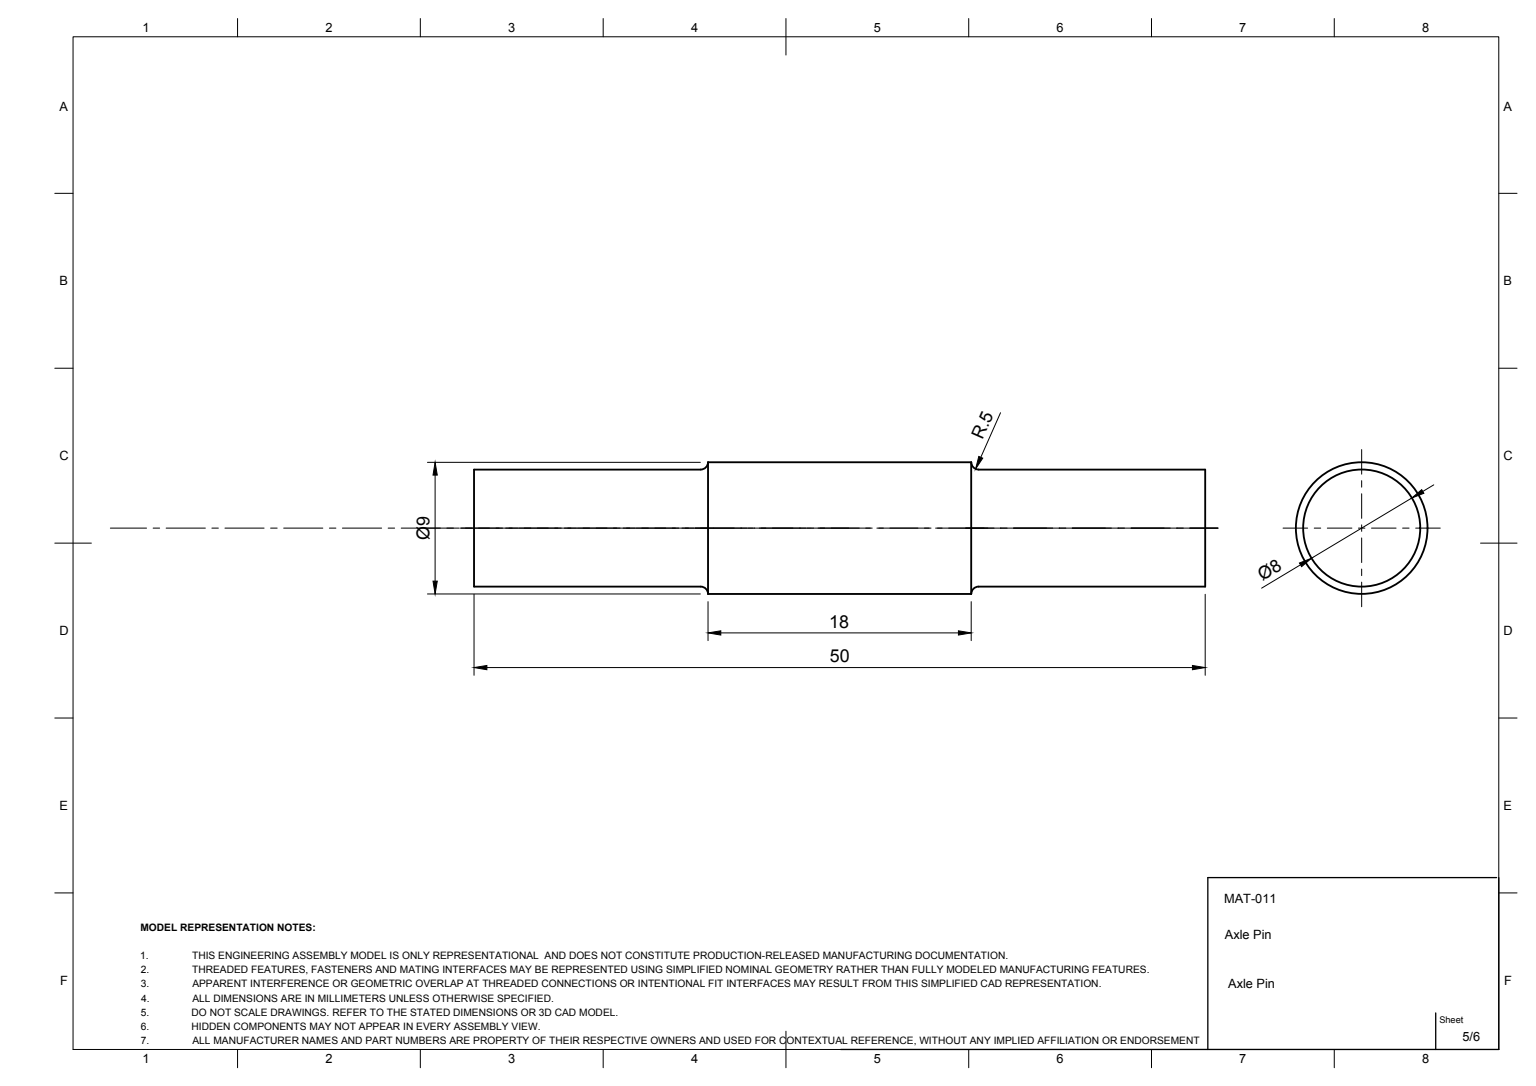
ISO-10303-21;
HEADER;
/* Generated by software containing ST-Developer
 * from STEP Tools, Inc. (www.steptools.com) 
 */

FILE_DESCRIPTION(
/* description */ ('STEP AP214'),
/* implementation_level */ '2;1');

FILE_NAME(
/* name */ 'Axle Pin.step',
/* time_stamp */ '2026-11-14T05:56:09-08:00',
/* author */ (''),
/* organization */ (''),
/* preprocessor_version */ 'ST-DEVELOPER v20.2',
/* originating_system */ 'Autodesk Translation Framework v15.17.0.0',
/* authorisation */ '');

FILE_SCHEMA (('AUTOMOTIVE_DESIGN { 1 0 10303 214 3 1 1 }'));
ENDSEC;

DATA;
#10=MECHANICAL_DESIGN_GEOMETRIC_PRESENTATION_REPRESENTATION('',(#104),#3207);
#92=SHAPE_REPRESENTATION_RELATIONSHIP('SRR','None',#3244,#98);
#98=ADVANCED_BREP_SHAPE_REPRESENTATION('',(#110),#3203);
#104=STYLED_ITEM('',(#3281),#110);
#110=MANIFOLD_SOLID_BREP('Body1',#1282);
#131=PLANE('',#1414);
#132=PLANE('',#1415);
#184=LINE('',#2091,#251);
#185=LINE('',#2093,#252);
#186=LINE('',#2096,#253);
#251=VECTOR('',#1666,4.);
#252=VECTOR('',#1669,4.5);
#253=VECTOR('',#1672,4.);
#290=CYLINDRICAL_SURFACE('',#1409,4.);
#291=CYLINDRICAL_SURFACE('',#1411,4.5);
#292=CYLINDRICAL_SURFACE('',#1412,4.);
#370=FACE_OUTER_BOUND('',#451,.T.);
#371=FACE_OUTER_BOUND('',#452,.T.);
#372=FACE_OUTER_BOUND('',#453,.T.);
#373=FACE_OUTER_BOUND('',#454,.T.);
#374=FACE_OUTER_BOUND('',#455,.T.);
#375=FACE_OUTER_BOUND('',#456,.T.);
#376=FACE_OUTER_BOUND('',#457,.T.);
#451=EDGE_LOOP('',(#965,#966,#967,#968));
#452=EDGE_LOOP('',(#969,#970,#971,#972,#973,#974));
#453=EDGE_LOOP('',(#975,#976,#977,#978,#979));
#454=EDGE_LOOP('',(#980,#981,#982,#983,#984));
#455=EDGE_LOOP('',(#985,#986,#987,#988));
#456=EDGE_LOOP('',(#989));
#457=EDGE_LOOP('',(#990));
#535=CIRCLE('',#1400,4.5);
#536=CIRCLE('',#1401,0.5);
#537=CIRCLE('',#1402,4.);
#538=CIRCLE('',#1404,4.5);
#539=CIRCLE('',#1405,0.5);
#540=CIRCLE('',#1406,4.);
#541=CIRCLE('',#1407,4.);
#542=CIRCLE('',#1408,4.5);
#543=CIRCLE('',#1410,4.);
#544=CIRCLE('',#1413,4.);
#619=VERTEX_POINT('',#2073);
#620=VERTEX_POINT('',#2075);
#621=VERTEX_POINT('',#2079);
#622=VERTEX_POINT('',#2080);
#623=VERTEX_POINT('',#2082);
#624=VERTEX_POINT('',#2084);
#625=VERTEX_POINT('',#2089);
#626=VERTEX_POINT('',#2095);
#746=EDGE_CURVE('',#619,#619,#535,.T.);
#747=EDGE_CURVE('',#619,#620,#536,.T.);
#748=EDGE_CURVE('',#620,#620,#537,.T.);
#749=EDGE_CURVE('',#621,#622,#538,.T.);
#750=EDGE_CURVE('',#622,#623,#539,.T.);
#751=EDGE_CURVE('',#624,#623,#540,.T.);
#752=EDGE_CURVE('',#623,#624,#541,.T.);
#753=EDGE_CURVE('',#622,#621,#542,.T.);
#754=EDGE_CURVE('',#625,#625,#543,.T.);
#755=EDGE_CURVE('',#625,#624,#184,.T.);
#756=EDGE_CURVE('',#621,#619,#185,.T.);
#757=EDGE_CURVE('',#620,#626,#186,.T.);
#758=EDGE_CURVE('',#626,#626,#544,.T.);
#965=ORIENTED_EDGE('',*,*,#746,.F.);
#966=ORIENTED_EDGE('',*,*,#747,.T.);
#967=ORIENTED_EDGE('',*,*,#748,.F.);
#968=ORIENTED_EDGE('',*,*,#747,.F.);
#969=ORIENTED_EDGE('',*,*,#749,.T.);
#970=ORIENTED_EDGE('',*,*,#750,.T.);
#971=ORIENTED_EDGE('',*,*,#751,.F.);
#972=ORIENTED_EDGE('',*,*,#752,.F.);
#973=ORIENTED_EDGE('',*,*,#750,.F.);
#974=ORIENTED_EDGE('',*,*,#753,.T.);
#975=ORIENTED_EDGE('',*,*,#754,.F.);
#976=ORIENTED_EDGE('',*,*,#755,.T.);
#977=ORIENTED_EDGE('',*,*,#751,.T.);
#978=ORIENTED_EDGE('',*,*,#752,.T.);
#979=ORIENTED_EDGE('',*,*,#755,.F.);
#980=ORIENTED_EDGE('',*,*,#749,.F.);
#981=ORIENTED_EDGE('',*,*,#756,.T.);
#982=ORIENTED_EDGE('',*,*,#746,.T.);
#983=ORIENTED_EDGE('',*,*,#756,.F.);
#984=ORIENTED_EDGE('',*,*,#753,.F.);
#985=ORIENTED_EDGE('',*,*,#748,.T.);
#986=ORIENTED_EDGE('',*,*,#757,.T.);
#987=ORIENTED_EDGE('',*,*,#758,.T.);
#988=ORIENTED_EDGE('',*,*,#757,.F.);
#989=ORIENTED_EDGE('',*,*,#758,.F.);
#990=ORIENTED_EDGE('',*,*,#754,.T.);
#1198=TOROIDAL_SURFACE('',#1399,4.5,0.5);
#1199=TOROIDAL_SURFACE('',#1403,4.5,0.5);
#1228=ADVANCED_FACE('',(#370),#1198,.F.);
#1229=ADVANCED_FACE('',(#371),#1199,.F.);
#1230=ADVANCED_FACE('',(#372),#290,.T.);
#1231=ADVANCED_FACE('',(#373),#291,.T.);
#1232=ADVANCED_FACE('',(#374),#292,.T.);
#1233=ADVANCED_FACE('',(#375),#131,.F.);
#1234=ADVANCED_FACE('',(#376),#132,.F.);
#1282=CLOSED_SHELL('',(#1228,#1229,#1230,#1231,#1232,#1233,#1234));
#1398=AXIS2_PLACEMENT_3D('',#2071,#1640,#1641);
#1399=AXIS2_PLACEMENT_3D('',#2072,#1642,#1643);
#1400=AXIS2_PLACEMENT_3D('',#2074,#1644,#1645);
#1401=AXIS2_PLACEMENT_3D('',#2076,#1646,#1647);
#1402=AXIS2_PLACEMENT_3D('',#2077,#1648,#1649);
#1403=AXIS2_PLACEMENT_3D('',#2078,#1650,#1651);
#1404=AXIS2_PLACEMENT_3D('',#2081,#1652,#1653);
#1405=AXIS2_PLACEMENT_3D('',#2083,#1654,#1655);
#1406=AXIS2_PLACEMENT_3D('',#2085,#1656,#1657);
#1407=AXIS2_PLACEMENT_3D('',#2086,#1658,#1659);
#1408=AXIS2_PLACEMENT_3D('',#2087,#1660,#1661);
#1409=AXIS2_PLACEMENT_3D('',#2088,#1662,#1663);
#1410=AXIS2_PLACEMENT_3D('',#2090,#1664,#1665);
#1411=AXIS2_PLACEMENT_3D('',#2092,#1667,#1668);
#1412=AXIS2_PLACEMENT_3D('',#2094,#1670,#1671);
#1413=AXIS2_PLACEMENT_3D('',#2097,#1673,#1674);
#1414=AXIS2_PLACEMENT_3D('',#2098,#1675,#1676);
#1415=AXIS2_PLACEMENT_3D('',#2099,#1677,#1678);
#1640=DIRECTION('axis',(0.,0.,1.));
#1641=DIRECTION('refdir',(1.,0.,0.));
#1642=DIRECTION('center_axis',(-1.,0.,0.));
#1643=DIRECTION('ref_axis',(0.,0.,1.));
#1644=DIRECTION('center_axis',(-1.,0.,0.));
#1645=DIRECTION('ref_axis',(0.,0.,1.));
#1646=DIRECTION('center_axis',(0.,1.,-1.22464679914735E-16));
#1647=DIRECTION('ref_axis',(0.,-1.22464679914735E-16,-1.));
#1648=DIRECTION('center_axis',(1.,0.,0.));
#1649=DIRECTION('ref_axis',(0.,0.,1.));
#1650=DIRECTION('center_axis',(1.,0.,0.));
#1651=DIRECTION('ref_axis',(0.,0.,-1.));
#1652=DIRECTION('center_axis',(-1.,0.,0.));
#1653=DIRECTION('ref_axis',(0.,0.,1.));
#1654=DIRECTION('center_axis',(0.,1.,1.22464679914735E-16));
#1655=DIRECTION('ref_axis',(0.,-1.22464679914735E-16,1.));
#1656=DIRECTION('center_axis',(-1.,0.,0.));
#1657=DIRECTION('ref_axis',(0.,0.,-1.));
#1658=DIRECTION('center_axis',(-1.,0.,0.));
#1659=DIRECTION('ref_axis',(0.,0.,-1.));
#1660=DIRECTION('center_axis',(-1.,0.,0.));
#1661=DIRECTION('ref_axis',(0.,0.,1.));
#1662=DIRECTION('center_axis',(-1.,0.,0.));
#1663=DIRECTION('ref_axis',(0.,0.,1.));
#1664=DIRECTION('center_axis',(-1.,0.,0.));
#1665=DIRECTION('ref_axis',(0.,0.,1.));
#1666=DIRECTION('',(1.,0.,0.));
#1667=DIRECTION('center_axis',(-1.,0.,0.));
#1668=DIRECTION('ref_axis',(0.,0.,1.));
#1669=DIRECTION('',(1.,0.,0.));
#1670=DIRECTION('center_axis',(-1.,0.,0.));
#1671=DIRECTION('ref_axis',(0.,0.,1.));
#1672=DIRECTION('',(1.,0.,0.));
#1673=DIRECTION('center_axis',(-1.,0.,0.));
#1674=DIRECTION('ref_axis',(0.,0.,1.));
#1675=DIRECTION('center_axis',(-1.,0.,0.));
#1676=DIRECTION('ref_axis',(0.,0.,1.));
#1677=DIRECTION('center_axis',(1.,0.,0.));
#1678=DIRECTION('ref_axis',(0.,0.,-1.));
#2071=CARTESIAN_POINT('',(0.,0.,0.));
#2072=CARTESIAN_POINT('Origin',(9.5,0.,0.));
#2073=CARTESIAN_POINT('',(9.,-5.51091059616309E-16,-4.5));
#2074=CARTESIAN_POINT('Origin',(9.,0.,0.));
#2075=CARTESIAN_POINT('',(9.5,-4.89858719658941E-16,-4.));
#2076=CARTESIAN_POINT('Origin',(9.5,-5.51091059616309E-16,-4.5));
#2077=CARTESIAN_POINT('Origin',(9.5,0.,0.));
#2078=CARTESIAN_POINT('Origin',(-9.5,0.,0.));
#2079=CARTESIAN_POINT('',(-9.,5.51091059616309E-16,-4.5));
#2080=CARTESIAN_POINT('',(-9.,-5.51091059616309E-16,4.5));
#2081=CARTESIAN_POINT('Origin',(-9.,0.,0.));
#2082=CARTESIAN_POINT('',(-9.5,-4.89858719658941E-16,4.));
#2083=CARTESIAN_POINT('Origin',(-9.5,-5.51091059616309E-16,4.5));
#2084=CARTESIAN_POINT('',(-9.5,4.89858719658941E-16,-4.));
#2085=CARTESIAN_POINT('Origin',(-9.5,0.,0.));
#2086=CARTESIAN_POINT('Origin',(-9.5,0.,0.));
#2087=CARTESIAN_POINT('Origin',(-9.,0.,0.));
#2088=CARTESIAN_POINT('Origin',(-25.,0.,0.));
#2089=CARTESIAN_POINT('',(-25.,-4.89858719658941E-16,-4.));
#2090=CARTESIAN_POINT('Origin',(-25.,0.,0.));
#2091=CARTESIAN_POINT('',(-25.,-4.89858719658941E-16,-4.));
#2092=CARTESIAN_POINT('Origin',(-25.,0.,0.));
#2093=CARTESIAN_POINT('',(-25.,-5.51091059616309E-16,-4.5));
#2094=CARTESIAN_POINT('Origin',(-25.,0.,0.));
#2095=CARTESIAN_POINT('',(25.,-4.89858719658941E-16,-4.));
#2096=CARTESIAN_POINT('',(-25.,-4.89858719658941E-16,-4.));
#2097=CARTESIAN_POINT('Origin',(25.,0.,0.));
#2098=CARTESIAN_POINT('Origin',(25.,0.,0.));
#2099=CARTESIAN_POINT('Origin',(-25.,0.,0.));
#3195=UNCERTAINTY_MEASURE_WITH_UNIT(LENGTH_MEASURE(0.01),#3208,
'DISTANCE_ACCURACY_VALUE',
'Maximum model space distance between geometric entities at asserted c
onnectivities');
#3199=UNCERTAINTY_MEASURE_WITH_UNIT(LENGTH_MEASURE(0.01),#3208,
'DISTANCE_ACCURACY_VALUE',
'Maximum model space distance between geometric entities at asserted c
onnectivities');
#3203=(
GEOMETRIC_REPRESENTATION_CONTEXT(3)
GLOBAL_UNCERTAINTY_ASSIGNED_CONTEXT((#3195))
GLOBAL_UNIT_ASSIGNED_CONTEXT((#3208,#3210,#3211))
REPRESENTATION_CONTEXT('','3D')
);
#3207=(
GEOMETRIC_REPRESENTATION_CONTEXT(3)
GLOBAL_UNCERTAINTY_ASSIGNED_CONTEXT((#3199))
GLOBAL_UNIT_ASSIGNED_CONTEXT((#3208,#3210,#3211))
REPRESENTATION_CONTEXT('','3D')
);
#3208=(
LENGTH_UNIT()
NAMED_UNIT(*)
SI_UNIT(.MILLI.,.METRE.)
);
#3210=(
NAMED_UNIT(*)
PLANE_ANGLE_UNIT()
SI_UNIT($,.RADIAN.)
);
#3211=(
NAMED_UNIT(*)
SI_UNIT($,.STERADIAN.)
SOLID_ANGLE_UNIT()
);
#3215=SHAPE_DEFINITION_REPRESENTATION(#3222,#3244);
#3222=PRODUCT_DEFINITION_SHAPE('',$,#3252);
#3244=SHAPE_REPRESENTATION('',(#1398),#3203);
#3248=PRODUCT_DEFINITION_CONTEXT('part definition',#3271,'design');
#3252=PRODUCT_DEFINITION('Axle Pin','Axle Pin',#3259,#3248);
#3259=PRODUCT_DEFINITION_FORMATION('',$,#3276);
#3271=APPLICATION_CONTEXT(
'Core Data for Automotive Mechanical Design Process');
#3272=PRODUCT_CONTEXT('part definition',#3271,'mechanical');
#3276=PRODUCT('Axle Pin','Axle Pin',$,(#3272));
#3281=PRESENTATION_STYLE_ASSIGNMENT((#3285));
#3285=SURFACE_STYLE_USAGE(.BOTH.,#3289);
#3289=SURFACE_SIDE_STYLE('',(#3293));
#3293=SURFACE_STYLE_FILL_AREA(#3297);
#3297=FILL_AREA_STYLE('Opaque(97,158,199)',(#3301));
#3301=FILL_AREA_STYLE_COLOUR('Opaque(97,158,199)',#3305);
#3305=COLOUR_RGB('Opaque(97,158,199)',0.380392156862745,0.619607843137255,
0.780392156862745);
ENDSEC;
END-ISO-10303-21;
